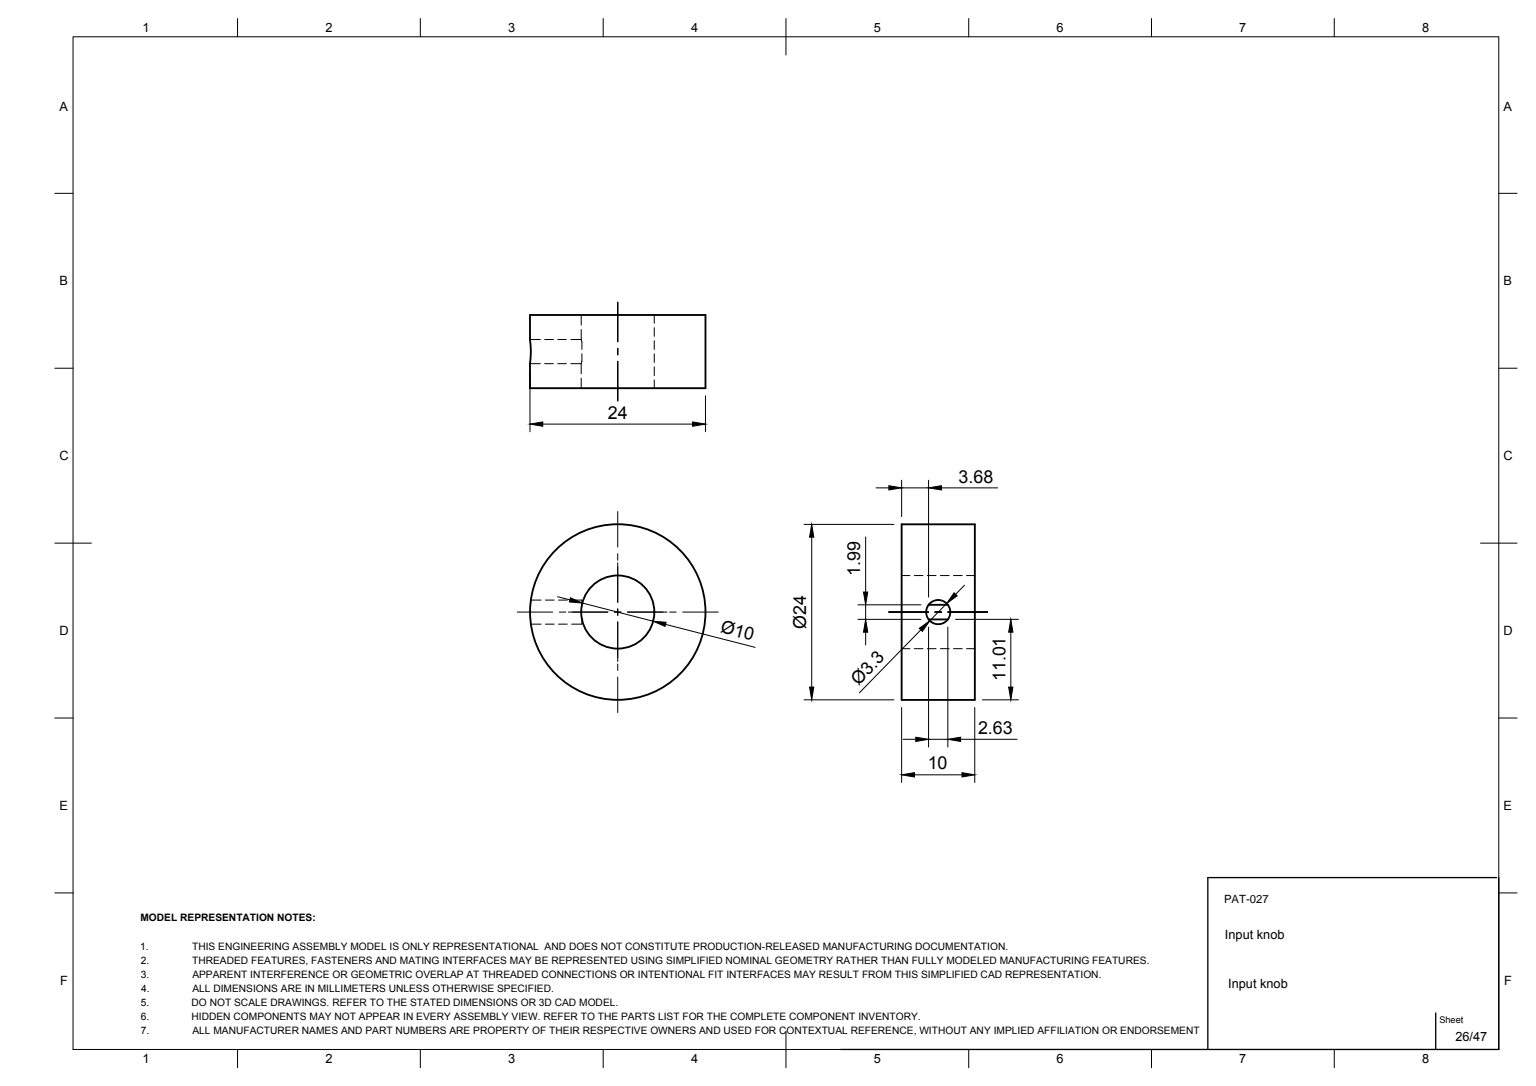
ISO-10303-21;
HEADER;
/* Generated by software containing ST-Developer
 * from STEP Tools, Inc. (www.steptools.com) 
 */

FILE_DESCRIPTION(
/* description */ ('Crank-driven oscillating fan base (mechanism only)'),

/* implementation_level */ '2;1');

FILE_NAME(
/* name */ 'Input knob.step',
/* time_stamp */ '2026-10-28T03:25:00-07:00',
/* author */ (''),
/* organization */ (''),
/* preprocessor_version */ 'ST-DEVELOPER v20.2',
/* originating_system */ 'Autodesk Translation Framework v15.17.0.0',
/* authorisation */ '');

FILE_SCHEMA (('AUTOMOTIVE_DESIGN { 1 0 10303 214 3 1 1 }'));
ENDSEC;

DATA;
#10=MECHANICAL_DESIGN_GEOMETRIC_PRESENTATION_REPRESENTATION('',(#463),#11916);
#347=B_SPLINE_CURVE_WITH_KNOTS('',3,(#10948,#10949,#10950,#10951,#10952,
#10953,#10954,#10955,#10956,#10957),.UNSPECIFIED.,.F.,.F.,(4,2,2,2,4),(0.649292020015383,
0.689320963667327,0.7519713082482,0.814621652829073,0.854650596481017),
 .UNSPECIFIED.);
#348=B_SPLINE_CURVE_WITH_KNOTS('',3,(#10961,#10962,#10963,#10964,#10965,
#10966),.UNSPECIFIED.,.F.,.F.,(4,2,4),(0.2506571027494,0.313307447330273,
0.353336390982217),.UNSPECIFIED.);
#349=B_SPLINE_CURVE_WITH_KNOTS('',3,(#10970,#10971,#10972,#10973,#10974,
#10975,#10976,#10977,#10978,#10979,#10980,#10981,#10982,#10983,#10984,#10985,
#10986,#10987,#10988,#10989,#10990,#10991,#10992,#10993,#10994,#10995),
 .UNSPECIFIED.,.F.,.F.,(4,2,2,2,2,2,2,2,2,2,2,2,4),(0.,0.0622384309821294,
0.124476861964259,0.186714529331343,0.248952196698428,0.311189864065512,
0.373427531432596,0.435665962414726,0.497904393396855,0.560142824378985,
0.622381255361114,0.684618922728198,0.746856590095283),.UNSPECIFIED.);
#350=B_SPLINE_CURVE_WITH_KNOTS('',3,(#10996,#10997,#10998,#10999,#11000,
#11001,#11002,#11003,#11004,#11005),.UNSPECIFIED.,.F.,.F.,(4,2,2,2,4),(0.746856590095283,
0.809094257462367,0.871331924829452,0.933570355811581,0.99580878679371),
 .UNSPECIFIED.);
#351=B_SPLINE_CURVE_WITH_KNOTS('',3,(#11006,#11007,#11008,#11009,#11010,
#11011),.UNSPECIFIED.,.F.,.F.,(4,2,4),(0.147977814516583,0.188006758168527,
0.2506571027494),.UNSPECIFIED.);
#375=SHAPE_REPRESENTATION_RELATIONSHIP('SRR','None',#12101,#415);
#415=ADVANCED_BREP_SHAPE_REPRESENTATION('',(#510),#11892);
#463=STYLED_ITEM('',(#12361),#510);
#510=MANIFOLD_SOLID_BREP('Body1',#6094);
#630=FACE_BOUND('',#1570,.T.);
#631=FACE_BOUND('',#1572,.T.);
#632=FACE_BOUND('',#1574,.T.);
#633=FACE_BOUND('',#1576,.T.);
#786=PLANE('',#7027);
#787=PLANE('',#7031);
#788=PLANE('',#7038);
#789=PLANE('',#7039);
#1091=FACE_OUTER_BOUND('',#1566,.T.);
#1092=FACE_OUTER_BOUND('',#1567,.T.);
#1093=FACE_OUTER_BOUND('',#1568,.T.);
#1094=FACE_OUTER_BOUND('',#1569,.T.);
#1095=FACE_OUTER_BOUND('',#1571,.T.);
#1096=FACE_OUTER_BOUND('',#1573,.T.);
#1097=FACE_OUTER_BOUND('',#1575,.T.);
#1566=EDGE_LOOP('',(#4926,#4927));
#1567=EDGE_LOOP('',(#4928,#4929,#4930,#4931,#4932,#4933,#4934,#4935,#4936));
#1568=EDGE_LOOP('',(#4937,#4938));
#1569=EDGE_LOOP('',(#4939,#4940,#4941,#4942));
#1570=EDGE_LOOP('',(#4943,#4944,#4945,#4946,#4947));
#1571=EDGE_LOOP('',(#4948,#4949,#4950,#4951));
#1572=EDGE_LOOP('',(#4952,#4953));
#1573=EDGE_LOOP('',(#4954));
#1574=EDGE_LOOP('',(#4955));
#1575=EDGE_LOOP('',(#4956));
#1576=EDGE_LOOP('',(#4957));
#1961=LINE('',#10944,#2294);
#1962=LINE('',#10968,#2295);
#1963=LINE('',#11013,#2296);
#1964=LINE('',#11018,#2297);
#1965=LINE('',#11024,#2298);
#2294=VECTOR('',#8512,1.);
#2295=VECTOR('',#8519,0.165);
#2296=VECTOR('',#8522,1.);
#2297=VECTOR('',#8527,0.5);
#2298=VECTOR('',#8534,1.2);
#2699=CIRCLE('',#7028,0.165);
#2700=CIRCLE('',#7030,0.165);
#2701=CIRCLE('',#7033,0.5);
#2702=CIRCLE('',#7034,0.5);
#2703=CIRCLE('',#7036,1.2);
#2704=CIRCLE('',#7037,1.2);
#3125=VERTEX_POINT('',#10942);
#3126=VERTEX_POINT('',#10943);
#3127=VERTEX_POINT('',#10947);
#3128=VERTEX_POINT('',#10958);
#3129=VERTEX_POINT('',#10960);
#3130=VERTEX_POINT('',#10967);
#3131=VERTEX_POINT('',#10969);
#3132=VERTEX_POINT('',#11015);
#3133=VERTEX_POINT('',#11017);
#3134=VERTEX_POINT('',#11021);
#3135=VERTEX_POINT('',#11023);
#3758=EDGE_CURVE('',#3125,#3126,#1961,.T.);
#3759=EDGE_CURVE('',#3125,#3126,#2699,.T.);
#3760=EDGE_CURVE('',#3127,#3125,#347,.T.);
#3761=EDGE_CURVE('',#3128,#3127,#2700,.T.);
#3762=EDGE_CURVE('',#3129,#3128,#348,.T.);
#3763=EDGE_CURVE('',#3129,#3130,#1962,.T.);
#3764=EDGE_CURVE('',#3131,#3130,#349,.T.);
#3765=EDGE_CURVE('',#3130,#3131,#350,.T.);
#3766=EDGE_CURVE('',#3126,#3129,#351,.T.);
#3767=EDGE_CURVE('',#3128,#3127,#1963,.T.);
#3768=EDGE_CURVE('',#3132,#3132,#2701,.T.);
#3769=EDGE_CURVE('',#3132,#3133,#1964,.T.);
#3770=EDGE_CURVE('',#3133,#3133,#2702,.T.);
#3771=EDGE_CURVE('',#3134,#3134,#2703,.T.);
#3772=EDGE_CURVE('',#3134,#3135,#1965,.T.);
#3773=EDGE_CURVE('',#3135,#3135,#2704,.T.);
#4926=ORIENTED_EDGE('',*,*,#3758,.F.);
#4927=ORIENTED_EDGE('',*,*,#3759,.T.);
#4928=ORIENTED_EDGE('',*,*,#3760,.F.);
#4929=ORIENTED_EDGE('',*,*,#3761,.F.);
#4930=ORIENTED_EDGE('',*,*,#3762,.F.);
#4931=ORIENTED_EDGE('',*,*,#3763,.T.);
#4932=ORIENTED_EDGE('',*,*,#3764,.F.);
#4933=ORIENTED_EDGE('',*,*,#3765,.F.);
#4934=ORIENTED_EDGE('',*,*,#3763,.F.);
#4935=ORIENTED_EDGE('',*,*,#3766,.F.);
#4936=ORIENTED_EDGE('',*,*,#3759,.F.);
#4937=ORIENTED_EDGE('',*,*,#3767,.F.);
#4938=ORIENTED_EDGE('',*,*,#3761,.T.);
#4939=ORIENTED_EDGE('',*,*,#3768,.F.);
#4940=ORIENTED_EDGE('',*,*,#3769,.T.);
#4941=ORIENTED_EDGE('',*,*,#3770,.T.);
#4942=ORIENTED_EDGE('',*,*,#3769,.F.);
#4943=ORIENTED_EDGE('',*,*,#3766,.T.);
#4944=ORIENTED_EDGE('',*,*,#3762,.T.);
#4945=ORIENTED_EDGE('',*,*,#3767,.T.);
#4946=ORIENTED_EDGE('',*,*,#3760,.T.);
#4947=ORIENTED_EDGE('',*,*,#3758,.T.);
#4948=ORIENTED_EDGE('',*,*,#3771,.F.);
#4949=ORIENTED_EDGE('',*,*,#3772,.T.);
#4950=ORIENTED_EDGE('',*,*,#3773,.T.);
#4951=ORIENTED_EDGE('',*,*,#3772,.F.);
#4952=ORIENTED_EDGE('',*,*,#3764,.T.);
#4953=ORIENTED_EDGE('',*,*,#3765,.T.);
#4954=ORIENTED_EDGE('',*,*,#3771,.T.);
#4955=ORIENTED_EDGE('',*,*,#3768,.T.);
#4956=ORIENTED_EDGE('',*,*,#3773,.F.);
#4957=ORIENTED_EDGE('',*,*,#3770,.F.);
#5632=CYLINDRICAL_SURFACE('',#7029,0.165);
#5633=CYLINDRICAL_SURFACE('',#7032,0.5);
#5634=CYLINDRICAL_SURFACE('',#7035,1.2);
#5897=ADVANCED_FACE('',(#1091),#786,.T.);
#5898=ADVANCED_FACE('',(#1092),#5632,.F.);
#5899=ADVANCED_FACE('',(#1093),#787,.T.);
#5900=ADVANCED_FACE('',(#1094,#630),#5633,.F.);
#5901=ADVANCED_FACE('',(#1095,#631),#5634,.T.);
#5902=ADVANCED_FACE('',(#1096,#632),#788,.T.);
#5903=ADVANCED_FACE('',(#1097,#633),#789,.F.);
#6094=CLOSED_SHELL('',(#5897,#5898,#5899,#5900,#5901,#5902,#5903));
#7026=AXIS2_PLACEMENT_3D('',#10940,#8508,#8509);
#7027=AXIS2_PLACEMENT_3D('',#10941,#8510,#8511);
#7028=AXIS2_PLACEMENT_3D('',#10945,#8513,#8514);
#7029=AXIS2_PLACEMENT_3D('',#10946,#8515,#8516);
#7030=AXIS2_PLACEMENT_3D('',#10959,#8517,#8518);
#7031=AXIS2_PLACEMENT_3D('',#11012,#8520,#8521);
#7032=AXIS2_PLACEMENT_3D('',#11014,#8523,#8524);
#7033=AXIS2_PLACEMENT_3D('',#11016,#8525,#8526);
#7034=AXIS2_PLACEMENT_3D('',#11019,#8528,#8529);
#7035=AXIS2_PLACEMENT_3D('',#11020,#8530,#8531);
#7036=AXIS2_PLACEMENT_3D('',#11022,#8532,#8533);
#7037=AXIS2_PLACEMENT_3D('',#11025,#8535,#8536);
#7038=AXIS2_PLACEMENT_3D('',#11026,#8537,#8538);
#7039=AXIS2_PLACEMENT_3D('',#11027,#8539,#8540);
#8508=DIRECTION('axis',(0.,0.,1.));
#8509=DIRECTION('refdir',(1.,0.,0.));
#8510=DIRECTION('center_axis',(1.,0.,0.));
#8511=DIRECTION('ref_axis',(0.,0.,-1.));
#8512=DIRECTION('',(0.,0.,1.));
#8513=DIRECTION('center_axis',(1.,0.,0.));
#8514=DIRECTION('ref_axis',(0.,0.,-1.));
#8515=DIRECTION('center_axis',(1.,0.,0.));
#8516=DIRECTION('ref_axis',(0.,0.,-1.));
#8517=DIRECTION('center_axis',(1.,0.,0.));
#8518=DIRECTION('ref_axis',(0.,0.,-1.));
#8519=DIRECTION('',(1.,0.,0.));
#8520=DIRECTION('center_axis',(1.,0.,0.));
#8521=DIRECTION('ref_axis',(0.,0.,-1.));
#8522=DIRECTION('',(0.,0.,-1.));
#8523=DIRECTION('center_axis',(0.,0.,1.));
#8524=DIRECTION('ref_axis',(1.,0.,0.));
#8525=DIRECTION('center_axis',(0.,0.,-1.));
#8526=DIRECTION('ref_axis',(1.,0.,0.));
#8527=DIRECTION('',(0.,0.,-1.));
#8528=DIRECTION('center_axis',(0.,0.,-1.));
#8529=DIRECTION('ref_axis',(1.,0.,0.));
#8530=DIRECTION('center_axis',(0.,0.,1.));
#8531=DIRECTION('ref_axis',(1.,0.,0.));
#8532=DIRECTION('center_axis',(0.,0.,1.));
#8533=DIRECTION('ref_axis',(1.,0.,0.));
#8534=DIRECTION('',(0.,0.,-1.));
#8535=DIRECTION('center_axis',(0.,0.,1.));
#8536=DIRECTION('ref_axis',(1.,0.,0.));
#8537=DIRECTION('center_axis',(0.,0.,1.));
#8538=DIRECTION('ref_axis',(1.,0.,0.));
#8539=DIRECTION('center_axis',(0.,0.,1.));
#8540=DIRECTION('ref_axis',(1.,0.,0.));
#10940=CARTESIAN_POINT('',(0.,0.,0.));
#10941=CARTESIAN_POINT('Origin',(0.49,0.,7.5));
#10942=CARTESIAN_POINT('',(0.49,0.0994987437106618,7.36837553418912));
#10943=CARTESIAN_POINT('',(0.49,0.0994987437106618,7.63162446581088));
#10944=CARTESIAN_POINT('',(0.49,0.0994987437106618,7.));
#10945=CARTESIAN_POINT('Origin',(0.49,0.,7.5));
#10946=CARTESIAN_POINT('Origin',(0.49,0.,7.5));
#10947=CARTESIAN_POINT('',(0.49,-0.0994987437106618,7.36837553418912));
#10948=CARTESIAN_POINT('Ctrl Pts',(0.49,-0.0994987437106616,7.36837553418912));
#10949=CARTESIAN_POINT('Ctrl Pts',(0.492216618113534,-0.0885825970828194,
7.36012370297415));
#10950=CARTESIAN_POINT('Ctrl Pts',(0.4943120869024,-0.0763322372136367,
7.35304490097489));
#10951=CARTESIAN_POINT('Ctrl Pts',(0.498563258730391,-0.0430544276449475,
7.33920540953364));
#10952=CARTESIAN_POINT('Ctrl Pts',(0.5,-0.0208834481936244,7.335));
#10953=CARTESIAN_POINT('Ctrl Pts',(0.5,0.0208834481936244,7.335));
#10954=CARTESIAN_POINT('Ctrl Pts',(0.498563258730391,0.0430544276449475,
7.33920540953364));
#10955=CARTESIAN_POINT('Ctrl Pts',(0.4943120869024,0.0763322372136367,7.3530449009749));
#10956=CARTESIAN_POINT('Ctrl Pts',(0.492216618113534,0.0885825970828194,
7.36012370297415));
#10957=CARTESIAN_POINT('Ctrl Pts',(0.49,0.0994987437106616,7.36837553418912));
#10958=CARTESIAN_POINT('',(0.49,-0.0994987437106618,7.63162446581088));
#10959=CARTESIAN_POINT('Origin',(0.49,0.,7.5));
#10960=CARTESIAN_POINT('',(0.5,3.77445171484879E-18,7.665));
#10961=CARTESIAN_POINT('Ctrl Pts',(0.5,-3.46944695195361E-18,7.665));
#10962=CARTESIAN_POINT('Ctrl Pts',(0.5,-0.0208834481936244,7.665));
#10963=CARTESIAN_POINT('Ctrl Pts',(0.498563258730391,-0.0430544276449474,
7.66079459046636));
#10964=CARTESIAN_POINT('Ctrl Pts',(0.4943120869024,-0.0763322372136367,
7.6469550990251));
#10965=CARTESIAN_POINT('Ctrl Pts',(0.492216618113534,-0.0885825970828193,
7.63987629702585));
#10966=CARTESIAN_POINT('Ctrl Pts',(0.49,-0.0994987437106615,7.63162446581088));
#10967=CARTESIAN_POINT('',(1.2,-2.02066721859313E-17,7.665));
#10968=CARTESIAN_POINT('',(0.49,-2.02066721859313E-17,7.665));
#10969=CARTESIAN_POINT('',(1.18860212013945,0.165,7.5));
#10970=CARTESIAN_POINT('Ctrl Pts',(1.18860212013945,0.165,7.5));
#10971=CARTESIAN_POINT('Ctrl Pts',(1.18860212013945,0.165,7.47925385633929));
#10972=CARTESIAN_POINT('Ctrl Pts',(1.18920136323583,0.16084848971883,7.45714308297918));
#10973=CARTESIAN_POINT('Ctrl Pts',(1.19135875380323,0.144001521209443,7.41649841577523));
#10974=CARTESIAN_POINT('Ctrl Pts',(1.19288497691659,0.131307482946399,7.39796224515484));
#10975=CARTESIAN_POINT('Ctrl Pts',(1.19574431960517,0.102037934403069,7.36869269661151));
#10976=CARTESIAN_POINT('Ctrl Pts',(1.1972642227448,0.0835016860163227,7.35599851755459));
#10977=CARTESIAN_POINT('Ctrl Pts',(1.19940712405299,0.0428567542973023,
7.33915144626121));
#10978=CARTESIAN_POINT('Ctrl Pts',(1.2,0.0207458891223615,7.335));
#10979=CARTESIAN_POINT('Ctrl Pts',(1.2,-0.0207458891223615,7.335));
#10980=CARTESIAN_POINT('Ctrl Pts',(1.19940712405299,-0.0428567542973023,
7.33915144626121));
#10981=CARTESIAN_POINT('Ctrl Pts',(1.1972642227448,-0.0835016860163228,
7.35599851755459));
#10982=CARTESIAN_POINT('Ctrl Pts',(1.19574431960517,-0.102037934403069,
7.36869269661151));
#10983=CARTESIAN_POINT('Ctrl Pts',(1.19288497691659,-0.131307482946399,
7.39796224515484));
#10984=CARTESIAN_POINT('Ctrl Pts',(1.19135875380323,-0.144001521209443,
7.41649841577523));
#10985=CARTESIAN_POINT('Ctrl Pts',(1.18920136323583,-0.16084848971883,7.45714308297918));
#10986=CARTESIAN_POINT('Ctrl Pts',(1.18860212013945,-0.165,7.47925385633929));
#10987=CARTESIAN_POINT('Ctrl Pts',(1.18860212013945,-0.165,7.52074614366071));
#10988=CARTESIAN_POINT('Ctrl Pts',(1.18920136323583,-0.16084848971883,7.54285691702082));
#10989=CARTESIAN_POINT('Ctrl Pts',(1.19135875380323,-0.144001521209443,
7.58350158422477));
#10990=CARTESIAN_POINT('Ctrl Pts',(1.19288497691659,-0.131307482946399,
7.60203775484516));
#10991=CARTESIAN_POINT('Ctrl Pts',(1.19574431960517,-0.102037934403069,
7.63130730338849));
#10992=CARTESIAN_POINT('Ctrl Pts',(1.1972642227448,-0.0835016860163227,
7.64400148244541));
#10993=CARTESIAN_POINT('Ctrl Pts',(1.19940712405299,-0.0428567542973023,
7.66084855373879));
#10994=CARTESIAN_POINT('Ctrl Pts',(1.2,-0.0207458891223615,7.665));
#10995=CARTESIAN_POINT('Ctrl Pts',(1.2,0.,7.665));
#10996=CARTESIAN_POINT('Ctrl Pts',(1.2,-4.85722573273506E-17,7.665));
#10997=CARTESIAN_POINT('Ctrl Pts',(1.2,0.0207458891223614,7.665));
#10998=CARTESIAN_POINT('Ctrl Pts',(1.19940712405299,0.0428567542973022,
7.66084855373879));
#10999=CARTESIAN_POINT('Ctrl Pts',(1.1972642227448,0.0835016860163227,7.64400148244541));
#11000=CARTESIAN_POINT('Ctrl Pts',(1.19574431960517,0.102037934403069,7.63130730338849));
#11001=CARTESIAN_POINT('Ctrl Pts',(1.19288497691659,0.131307482946399,7.60203775484516));
#11002=CARTESIAN_POINT('Ctrl Pts',(1.19135875380323,0.144001521209443,7.58350158422477));
#11003=CARTESIAN_POINT('Ctrl Pts',(1.18920136323583,0.16084848971883,7.54285691702082));
#11004=CARTESIAN_POINT('Ctrl Pts',(1.18860212013945,0.165,7.52074614366071));
#11005=CARTESIAN_POINT('Ctrl Pts',(1.18860212013945,0.165,7.5));
#11006=CARTESIAN_POINT('Ctrl Pts',(0.49,0.0994987437106614,7.63162446581088));
#11007=CARTESIAN_POINT('Ctrl Pts',(0.492216618113534,0.0885825970828193,
7.63987629702585));
#11008=CARTESIAN_POINT('Ctrl Pts',(0.4943120869024,0.0763322372136366,7.6469550990251));
#11009=CARTESIAN_POINT('Ctrl Pts',(0.498563258730391,0.0430544276449474,
7.66079459046636));
#11010=CARTESIAN_POINT('Ctrl Pts',(0.5,0.0208834481936243,7.665));
#11011=CARTESIAN_POINT('Ctrl Pts',(0.5,-5.55111512312578E-17,7.665));
#11012=CARTESIAN_POINT('Origin',(0.49,0.,7.5));
#11013=CARTESIAN_POINT('',(0.49,-0.0994987437106618,7.));
#11014=CARTESIAN_POINT('Origin',(0.,0.,7.));
#11015=CARTESIAN_POINT('',(-0.5,-6.12323399573677E-17,8.));
#11016=CARTESIAN_POINT('Origin',(0.,0.,8.));
#11017=CARTESIAN_POINT('',(-0.5,-6.12323399573677E-17,7.));
#11018=CARTESIAN_POINT('',(-0.5,-6.12323399573677E-17,7.));
#11019=CARTESIAN_POINT('Origin',(0.,0.,7.));
#11020=CARTESIAN_POINT('Origin',(0.,0.,7.));
#11021=CARTESIAN_POINT('',(-1.2,-1.46957615897682E-16,8.));
#11022=CARTESIAN_POINT('Origin',(0.,0.,8.));
#11023=CARTESIAN_POINT('',(-1.2,-1.46957615897682E-16,7.));
#11024=CARTESIAN_POINT('',(-1.2,-1.46957615897682E-16,7.));
#11025=CARTESIAN_POINT('Origin',(0.,0.,7.));
#11026=CARTESIAN_POINT('Origin',(0.,0.,8.));
#11027=CARTESIAN_POINT('Origin',(0.,0.,7.));
#11845=UNCERTAINTY_MEASURE_WITH_UNIT(LENGTH_MEASURE(0.001),#11917,
'DISTANCE_ACCURACY_VALUE',
'Maximum model space distance between geometric entities at asserted c
onnectivities');
#11869=UNCERTAINTY_MEASURE_WITH_UNIT(LENGTH_MEASURE(0.001),#11917,
'DISTANCE_ACCURACY_VALUE',
'Maximum model space distance between geometric entities at asserted c
onnectivities');
#11892=(
GEOMETRIC_REPRESENTATION_CONTEXT(3)
GLOBAL_UNCERTAINTY_ASSIGNED_CONTEXT((#11845))
GLOBAL_UNIT_ASSIGNED_CONTEXT((#11917,#11919,#11920))
REPRESENTATION_CONTEXT('','3D')
);
#11916=(
GEOMETRIC_REPRESENTATION_CONTEXT(3)
GLOBAL_UNCERTAINTY_ASSIGNED_CONTEXT((#11869))
GLOBAL_UNIT_ASSIGNED_CONTEXT((#11917,#11919,#11920))
REPRESENTATION_CONTEXT('','3D')
);
#11917=(
LENGTH_UNIT()
NAMED_UNIT(*)
SI_UNIT(.CENTI.,.METRE.)
);
#11919=(
NAMED_UNIT(*)
PLANE_ANGLE_UNIT()
SI_UNIT($,.RADIAN.)
);
#11920=(
NAMED_UNIT(*)
SI_UNIT($,.STERADIAN.)
SOLID_ANGLE_UNIT()
);
#11943=SHAPE_DEFINITION_REPRESENTATION(#11994,#12101);
#11994=PRODUCT_DEFINITION_SHAPE('',$,#12148);
#12101=SHAPE_REPRESENTATION('',(#7026),#11892);
#12125=PRODUCT_DEFINITION_CONTEXT('part definition',#12265,'design');
#12148=PRODUCT_DEFINITION('Input knob','Input knob',#12194,#12125);
#12194=PRODUCT_DEFINITION_FORMATION('',$,#12289);
#12265=APPLICATION_CONTEXT(
'Core Data for Automotive Mechanical Design Process');
#12266=PRODUCT_CONTEXT('part definition',#12265,'mechanical');
#12289=PRODUCT('Input knob','Input knob','Input knob',(#12266));
#12355=COLOUR_RGB('Light Blue',0.38,0.62,0.78);
#12356=FILL_AREA_STYLE_COLOUR('',#12355);
#12357=FILL_AREA_STYLE('',(#12356));
#12358=SURFACE_STYLE_FILL_AREA(#12357);
#12359=SURFACE_SIDE_STYLE('',(#12358));
#12360=SURFACE_STYLE_USAGE(.BOTH.,#12359);
#12361=PRESENTATION_STYLE_ASSIGNMENT((#12360));
ENDSEC;
END-ISO-10303-21;
